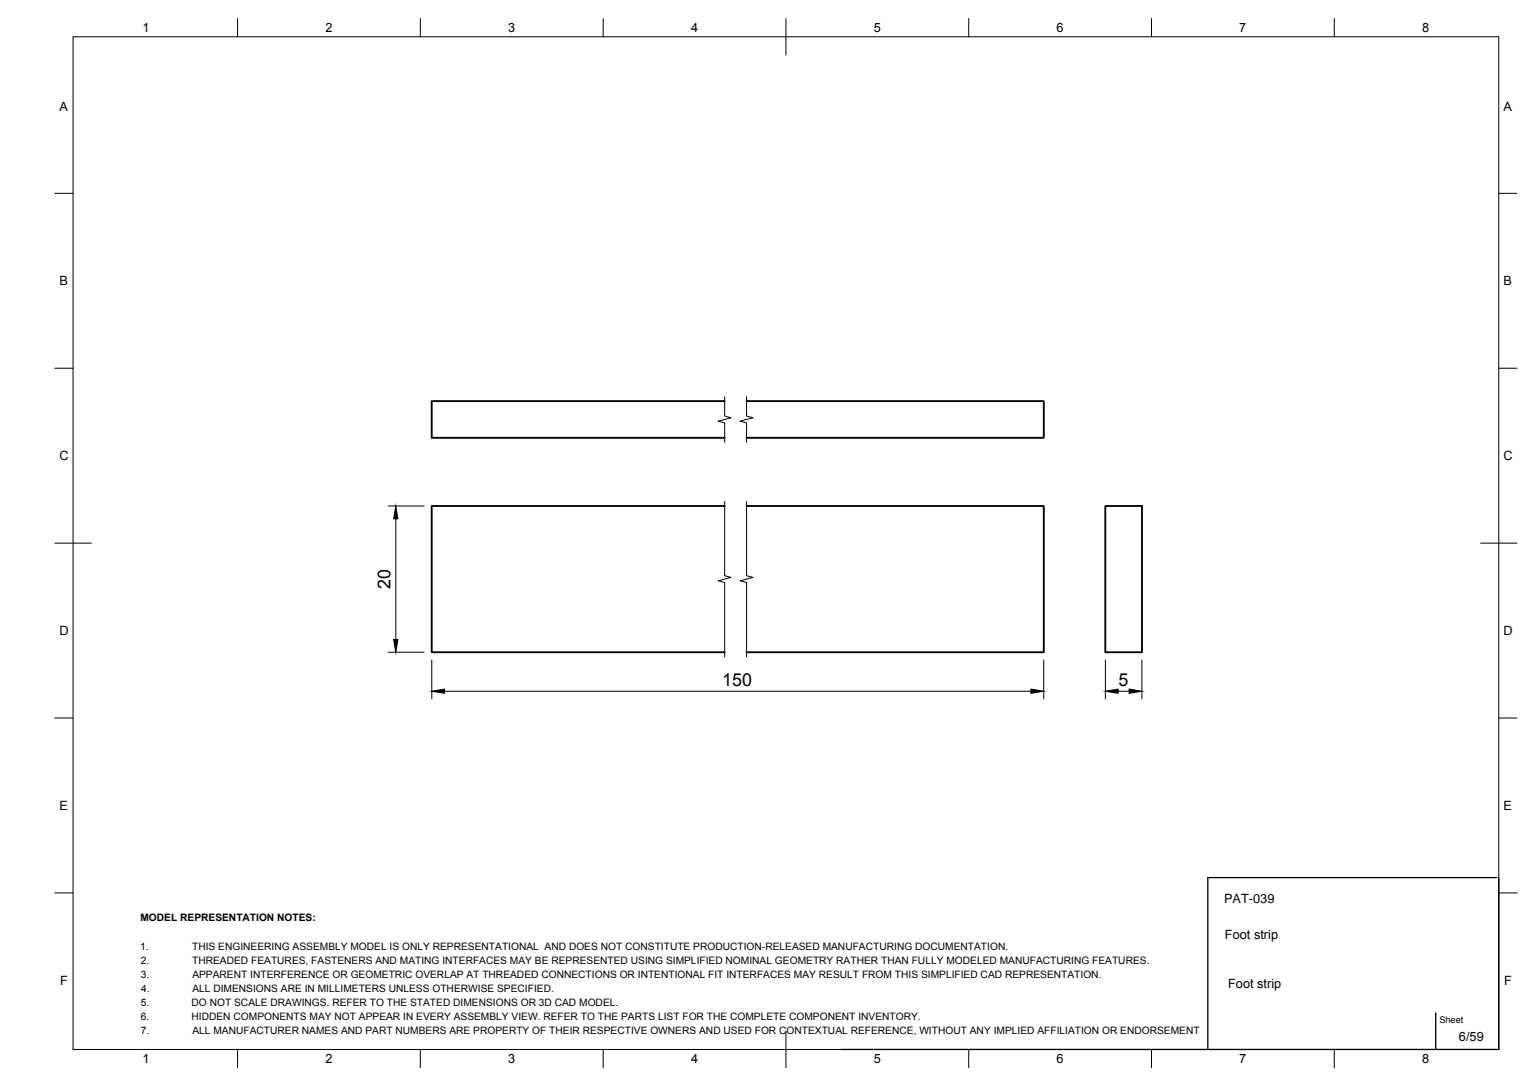
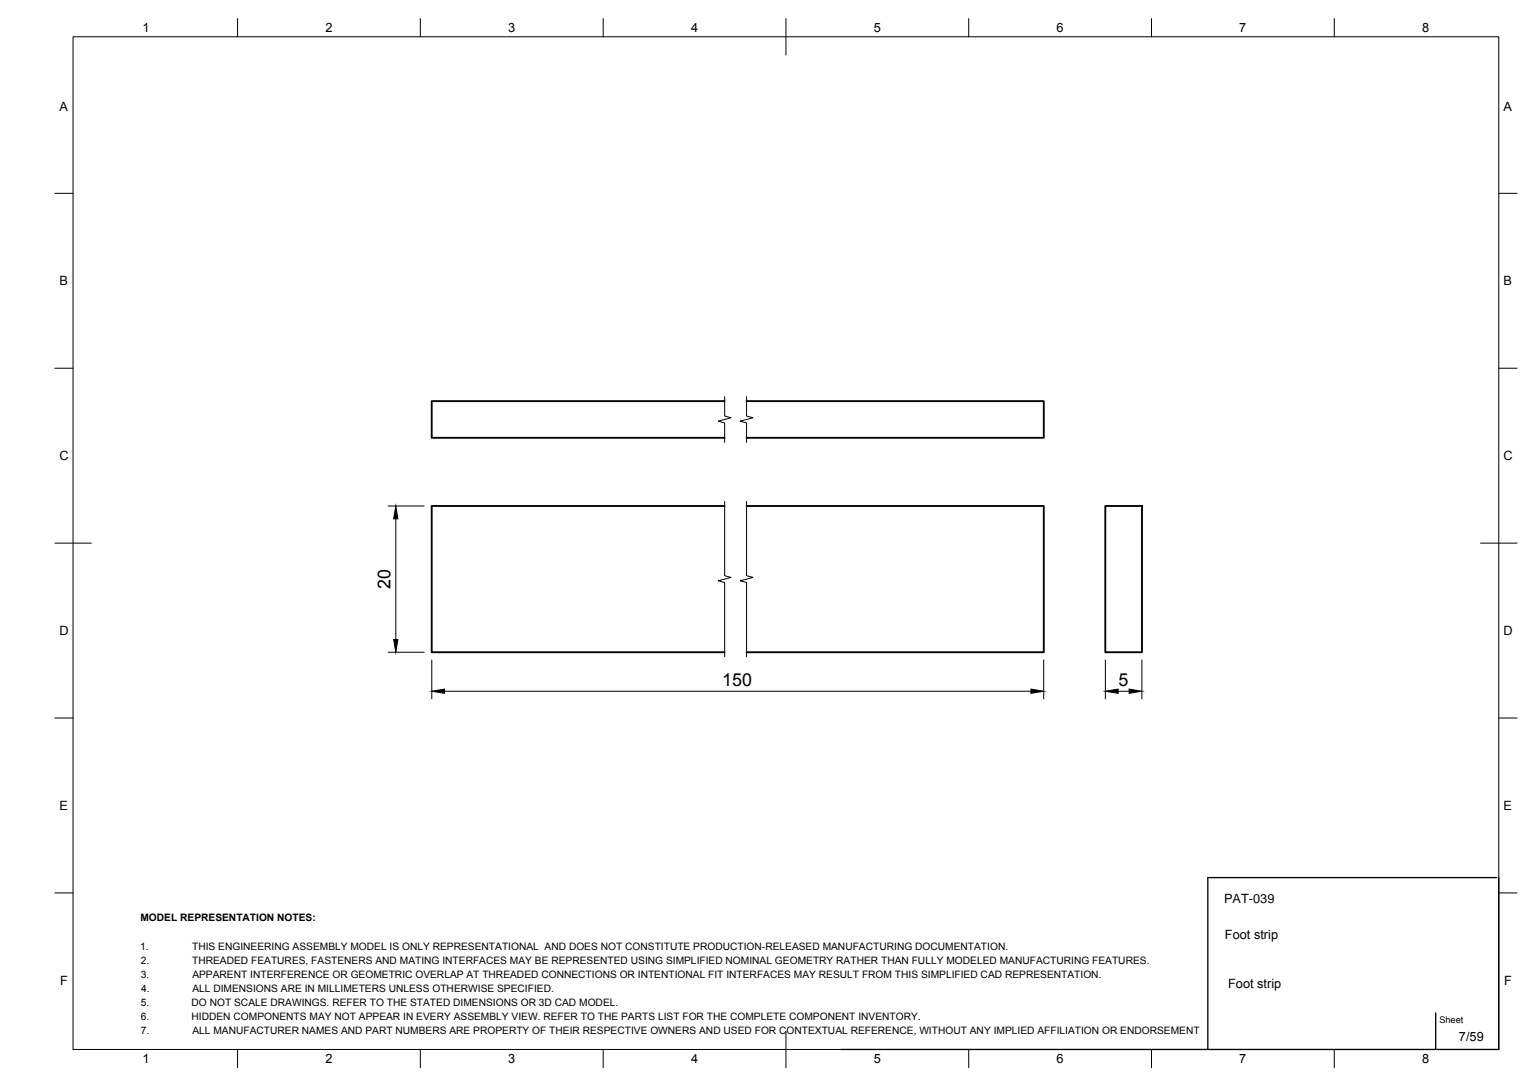
ISO-10303-21;
HEADER;
/* Generated by software containing ST-Developer
 * from STEP Tools, Inc. (www.steptools.com) 
 */

FILE_DESCRIPTION(
/* description */ ('Four-bar parallelogram arm'),
/* implementation_level */ '2;1');

FILE_NAME(
/* name */ 'Foot strip.step',
/* time_stamp */ '2026-10-28T03:24:55-07:00',
/* author */ (''),
/* organization */ (''),
/* preprocessor_version */ 'ST-DEVELOPER v20.2',
/* originating_system */ 'Autodesk Translation Framework v15.17.0.0',
/* authorisation */ '');

FILE_SCHEMA (('AUTOMOTIVE_DESIGN { 1 0 10303 214 3 1 1 }'));
ENDSEC;

DATA;
#10=MECHANICAL_DESIGN_GEOMETRIC_PRESENTATION_REPRESENTATION('',(#623),#14512);
#523=SHAPE_REPRESENTATION_RELATIONSHIP('SRR','None',#14744,#573);
#573=ADVANCED_BREP_SHAPE_REPRESENTATION('',(#681),#14459);
#623=STYLED_ITEM('',(#15073),#681);
#681=MANIFOLD_SOLID_BREP('Body1',#7327);
#1012=PLANE('',#7960);
#1013=PLANE('',#7961);
#1014=PLANE('',#7962);
#1015=PLANE('',#7963);
#1016=PLANE('',#7964);
#1017=PLANE('',#7965);
#1211=FACE_OUTER_BOUND('',#1639,.T.);
#1212=FACE_OUTER_BOUND('',#1640,.T.);
#1213=FACE_OUTER_BOUND('',#1641,.T.);
#1214=FACE_OUTER_BOUND('',#1642,.T.);
#1215=FACE_OUTER_BOUND('',#1643,.T.);
#1216=FACE_OUTER_BOUND('',#1644,.T.);
#1639=EDGE_LOOP('',(#5036,#5037,#5038,#5039));
#1640=EDGE_LOOP('',(#5040,#5041,#5042,#5043));
#1641=EDGE_LOOP('',(#5044,#5045,#5046,#5047));
#1642=EDGE_LOOP('',(#5048,#5049,#5050,#5051));
#1643=EDGE_LOOP('',(#5052,#5053,#5054,#5055));
#1644=EDGE_LOOP('',(#5056,#5057,#5058,#5059));
#2328=LINE('',#11485,#2722);
#2329=LINE('',#11487,#2723);
#2330=LINE('',#11489,#2724);
#2331=LINE('',#11490,#2725);
#2332=LINE('',#11493,#2726);
#2333=LINE('',#11495,#2727);
#2334=LINE('',#11496,#2728);
#2335=LINE('',#11499,#2729);
#2336=LINE('',#11501,#2730);
#2337=LINE('',#11502,#2731);
#2338=LINE('',#11504,#2732);
#2339=LINE('',#11505,#2733);
#2722=VECTOR('',#9032,1.);
#2723=VECTOR('',#9033,1.);
#2724=VECTOR('',#9034,1.);
#2725=VECTOR('',#9035,1.);
#2726=VECTOR('',#9038,1.);
#2727=VECTOR('',#9039,1.);
#2728=VECTOR('',#9040,1.);
#2729=VECTOR('',#9043,1.);
#2730=VECTOR('',#9044,1.);
#2731=VECTOR('',#9045,1.);
#2732=VECTOR('',#9048,1.);
#2733=VECTOR('',#9049,1.);
#3561=VERTEX_POINT('',#11483);
#3562=VERTEX_POINT('',#11484);
#3563=VERTEX_POINT('',#11486);
#3564=VERTEX_POINT('',#11488);
#3565=VERTEX_POINT('',#11492);
#3566=VERTEX_POINT('',#11494);
#3567=VERTEX_POINT('',#11498);
#3568=VERTEX_POINT('',#11500);
#4149=EDGE_CURVE('',#3561,#3562,#2328,.T.);
#4150=EDGE_CURVE('',#3562,#3563,#2329,.T.);
#4151=EDGE_CURVE('',#3564,#3563,#2330,.T.);
#4152=EDGE_CURVE('',#3561,#3564,#2331,.T.);
#4153=EDGE_CURVE('',#3565,#3561,#2332,.T.);
#4154=EDGE_CURVE('',#3566,#3564,#2333,.T.);
#4155=EDGE_CURVE('',#3565,#3566,#2334,.T.);
#4156=EDGE_CURVE('',#3567,#3565,#2335,.T.);
#4157=EDGE_CURVE('',#3568,#3566,#2336,.T.);
#4158=EDGE_CURVE('',#3567,#3568,#2337,.T.);
#4159=EDGE_CURVE('',#3562,#3567,#2338,.T.);
#4160=EDGE_CURVE('',#3563,#3568,#2339,.T.);
#5036=ORIENTED_EDGE('',*,*,#4149,.T.);
#5037=ORIENTED_EDGE('',*,*,#4150,.T.);
#5038=ORIENTED_EDGE('',*,*,#4151,.F.);
#5039=ORIENTED_EDGE('',*,*,#4152,.F.);
#5040=ORIENTED_EDGE('',*,*,#4153,.T.);
#5041=ORIENTED_EDGE('',*,*,#4152,.T.);
#5042=ORIENTED_EDGE('',*,*,#4154,.F.);
#5043=ORIENTED_EDGE('',*,*,#4155,.F.);
#5044=ORIENTED_EDGE('',*,*,#4156,.T.);
#5045=ORIENTED_EDGE('',*,*,#4155,.T.);
#5046=ORIENTED_EDGE('',*,*,#4157,.F.);
#5047=ORIENTED_EDGE('',*,*,#4158,.F.);
#5048=ORIENTED_EDGE('',*,*,#4159,.T.);
#5049=ORIENTED_EDGE('',*,*,#4158,.T.);
#5050=ORIENTED_EDGE('',*,*,#4160,.F.);
#5051=ORIENTED_EDGE('',*,*,#4150,.F.);
#5052=ORIENTED_EDGE('',*,*,#4160,.T.);
#5053=ORIENTED_EDGE('',*,*,#4157,.T.);
#5054=ORIENTED_EDGE('',*,*,#4154,.T.);
#5055=ORIENTED_EDGE('',*,*,#4151,.T.);
#5056=ORIENTED_EDGE('',*,*,#4159,.F.);
#5057=ORIENTED_EDGE('',*,*,#4149,.F.);
#5058=ORIENTED_EDGE('',*,*,#4153,.F.);
#5059=ORIENTED_EDGE('',*,*,#4156,.F.);
#6916=ADVANCED_FACE('',(#1211),#1012,.T.);
#6917=ADVANCED_FACE('',(#1212),#1013,.T.);
#6918=ADVANCED_FACE('',(#1213),#1014,.T.);
#6919=ADVANCED_FACE('',(#1214),#1015,.T.);
#6920=ADVANCED_FACE('',(#1215),#1016,.T.);
#6921=ADVANCED_FACE('',(#1216),#1017,.F.);
#7327=CLOSED_SHELL('',(#6916,#6917,#6918,#6919,#6920,#6921));
#7959=AXIS2_PLACEMENT_3D('',#11481,#9028,#9029);
#7960=AXIS2_PLACEMENT_3D('',#11482,#9030,#9031);
#7961=AXIS2_PLACEMENT_3D('',#11491,#9036,#9037);
#7962=AXIS2_PLACEMENT_3D('',#11497,#9041,#9042);
#7963=AXIS2_PLACEMENT_3D('',#11503,#9046,#9047);
#7964=AXIS2_PLACEMENT_3D('',#11506,#9050,#9051);
#7965=AXIS2_PLACEMENT_3D('',#11507,#9052,#9053);
#9028=DIRECTION('axis',(0.,0.,1.));
#9029=DIRECTION('refdir',(1.,0.,0.));
#9030=DIRECTION('center_axis',(0.,1.,0.));
#9031=DIRECTION('ref_axis',(-1.,0.,0.));
#9032=DIRECTION('',(-1.,0.,0.));
#9033=DIRECTION('',(0.,0.,1.));
#9034=DIRECTION('',(-1.,0.,0.));
#9035=DIRECTION('',(0.,0.,1.));
#9036=DIRECTION('center_axis',(1.,0.,0.));
#9037=DIRECTION('ref_axis',(0.,1.,0.));
#9038=DIRECTION('',(0.,1.,0.));
#9039=DIRECTION('',(0.,1.,0.));
#9040=DIRECTION('',(0.,0.,1.));
#9041=DIRECTION('center_axis',(0.,-1.,0.));
#9042=DIRECTION('ref_axis',(1.,0.,0.));
#9043=DIRECTION('',(1.,0.,0.));
#9044=DIRECTION('',(1.,0.,0.));
#9045=DIRECTION('',(0.,0.,1.));
#9046=DIRECTION('center_axis',(-1.,0.,0.));
#9047=DIRECTION('ref_axis',(0.,-1.,0.));
#9048=DIRECTION('',(0.,-1.,0.));
#9049=DIRECTION('',(0.,-1.,0.));
#9050=DIRECTION('center_axis',(0.,0.,1.));
#9051=DIRECTION('ref_axis',(1.,0.,0.));
#9052=DIRECTION('center_axis',(0.,0.,1.));
#9053=DIRECTION('ref_axis',(1.,0.,0.));
#11481=CARTESIAN_POINT('',(0.,0.,0.));
#11482=CARTESIAN_POINT('Origin',(-3.,10.,-0.5));
#11483=CARTESIAN_POINT('',(-3.,10.,-0.5));
#11484=CARTESIAN_POINT('',(-5.,10.,-0.5));
#11485=CARTESIAN_POINT('',(-3.,10.,-0.5));
#11486=CARTESIAN_POINT('',(-5.,10.,0.));
#11487=CARTESIAN_POINT('',(-5.,10.,-0.5));
#11488=CARTESIAN_POINT('',(-3.,10.,0.));
#11489=CARTESIAN_POINT('',(-3.,10.,0.));
#11490=CARTESIAN_POINT('',(-3.,10.,-0.5));
#11491=CARTESIAN_POINT('Origin',(-3.,-5.,-0.5));
#11492=CARTESIAN_POINT('',(-3.,-5.,-0.5));
#11493=CARTESIAN_POINT('',(-3.,-5.,-0.5));
#11494=CARTESIAN_POINT('',(-3.,-5.,0.));
#11495=CARTESIAN_POINT('',(-3.,-5.,0.));
#11496=CARTESIAN_POINT('',(-3.,-5.,-0.5));
#11497=CARTESIAN_POINT('Origin',(-5.,-5.,-0.5));
#11498=CARTESIAN_POINT('',(-5.,-5.,-0.5));
#11499=CARTESIAN_POINT('',(-5.,-5.,-0.5));
#11500=CARTESIAN_POINT('',(-5.,-5.,0.));
#11501=CARTESIAN_POINT('',(-5.,-5.,0.));
#11502=CARTESIAN_POINT('',(-5.,-5.,-0.5));
#11503=CARTESIAN_POINT('Origin',(-5.,10.,-0.5));
#11504=CARTESIAN_POINT('',(-5.,10.,-0.5));
#11505=CARTESIAN_POINT('',(-5.,10.,0.));
#11506=CARTESIAN_POINT('Origin',(-4.,2.5,0.));
#11507=CARTESIAN_POINT('Origin',(-4.,2.5,-0.5));
#14402=UNCERTAINTY_MEASURE_WITH_UNIT(LENGTH_MEASURE(0.001),#14513,
'DISTANCE_ACCURACY_VALUE',
'Maximum model space distance between geometric entities at asserted c
onnectivities');
#14455=UNCERTAINTY_MEASURE_WITH_UNIT(LENGTH_MEASURE(0.001),#14513,
'DISTANCE_ACCURACY_VALUE',
'Maximum model space distance between geometric entities at asserted c
onnectivities');
#14459=(
GEOMETRIC_REPRESENTATION_CONTEXT(3)
GLOBAL_UNCERTAINTY_ASSIGNED_CONTEXT((#14402))
GLOBAL_UNIT_ASSIGNED_CONTEXT((#14513,#14515,#14516))
REPRESENTATION_CONTEXT('','3D')
);
#14512=(
GEOMETRIC_REPRESENTATION_CONTEXT(3)
GLOBAL_UNCERTAINTY_ASSIGNED_CONTEXT((#14455))
GLOBAL_UNIT_ASSIGNED_CONTEXT((#14513,#14515,#14516))
REPRESENTATION_CONTEXT('','3D')
);
#14513=(
LENGTH_UNIT()
NAMED_UNIT(*)
SI_UNIT(.CENTI.,.METRE.)
);
#14515=(
NAMED_UNIT(*)
PLANE_ANGLE_UNIT()
SI_UNIT($,.RADIAN.)
);
#14516=(
NAMED_UNIT(*)
SI_UNIT($,.STERADIAN.)
SOLID_ANGLE_UNIT()
);
#14520=SHAPE_DEFINITION_REPRESENTATION(#14576,#14744);
#14576=PRODUCT_DEFINITION_SHAPE('',$,#14801);
#14744=SHAPE_REPRESENTATION('',(#7959),#14459);
#14797=PRODUCT_DEFINITION_CONTEXT('part definition',#14967,'design');
#14801=PRODUCT_DEFINITION('Foot strip','Foot strip',#14857,#14797);
#14857=PRODUCT_DEFINITION_FORMATION('',$,#14972);
#14967=APPLICATION_CONTEXT(
'Core Data for Automotive Mechanical Design Process');
#14968=PRODUCT_CONTEXT('part definition',#14967,'mechanical');
#14972=PRODUCT('Foot strip','Foot strip','Foot strip',(#14968));
#15067=COLOUR_RGB('Light Blue',0.38,0.62,0.78);
#15068=FILL_AREA_STYLE_COLOUR('',#15067);
#15069=FILL_AREA_STYLE('',(#15068));
#15070=SURFACE_STYLE_FILL_AREA(#15069);
#15071=SURFACE_SIDE_STYLE('',(#15070));
#15072=SURFACE_STYLE_USAGE(.BOTH.,#15071);
#15073=PRESENTATION_STYLE_ASSIGNMENT((#15072));
ENDSEC;
END-ISO-10303-21;
